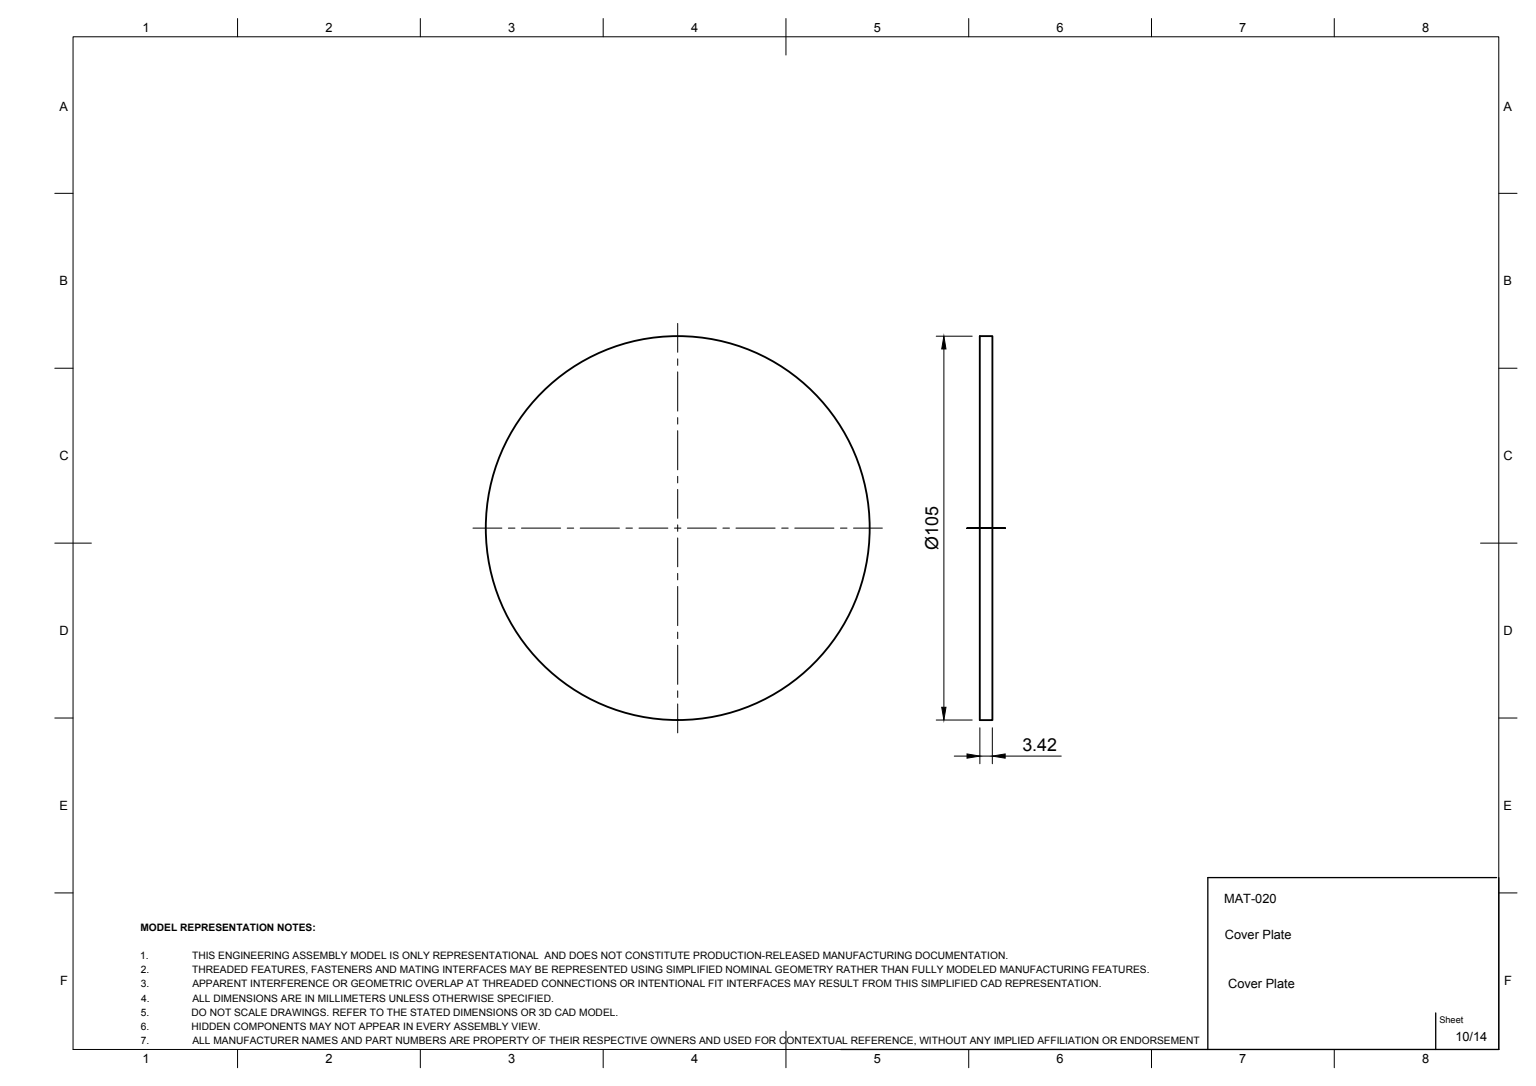
ISO-10303-21;
HEADER;
/* Generated by software containing ST-Developer
 * from STEP Tools, Inc. (www.steptools.com) 
 */

FILE_DESCRIPTION(
/* description */ ('STEP AP214'),
/* implementation_level */ '2;1');

FILE_NAME(
/* name */ 'Cover Plate.step',
/* time_stamp */ '2026-11-14T06:20:50-08:00',
/* author */ (''),
/* organization */ (''),
/* preprocessor_version */ 'ST-DEVELOPER v20.2',
/* originating_system */ 'Autodesk Translation Framework v15.17.0.0',
/* authorisation */ '');

FILE_SCHEMA (('AUTOMOTIVE_DESIGN { 1 0 10303 214 3 1 1 }'));
ENDSEC;

DATA;
#10=MECHANICAL_DESIGN_GEOMETRIC_PRESENTATION_REPRESENTATION('',(#961),#20658);
#422=PLANE('',#3970);
#423=PLANE('',#3971);
#592=LINE('',#20304,#785);
#785=VECTOR('',#4619,52.5);
#905=CYLINDRICAL_SURFACE('',#3967,52.5);
#937=SHAPE_REPRESENTATION_RELATIONSHIP('SRR','None',#20721,#949);
#949=ADVANCED_BREP_SHAPE_REPRESENTATION('',(#973),#20651);
#961=STYLED_ITEM('',(#20786),#973);
#973=MANIFOLD_SOLID_BREP('Body1',#3656);
#1126=FACE_OUTER_BOUND('',#1343,.T.);
#1127=FACE_OUTER_BOUND('',#1344,.T.);
#1128=FACE_OUTER_BOUND('',#1345,.T.);
#1343=EDGE_LOOP('',(#3200,#3201,#3202,#3203));
#1344=EDGE_LOOP('',(#3204));
#1345=EDGE_LOOP('',(#3205));
#1483=CIRCLE('',#3968,52.5);
#1484=CIRCLE('',#3969,52.5);
#1811=VERTEX_POINT('',#20301);
#1812=VERTEX_POINT('',#20303);
#2282=EDGE_CURVE('',#1811,#1811,#1483,.T.);
#2283=EDGE_CURVE('',#1811,#1812,#592,.T.);
#2284=EDGE_CURVE('',#1812,#1812,#1484,.T.);
#3200=ORIENTED_EDGE('',*,*,#2282,.T.);
#3201=ORIENTED_EDGE('',*,*,#2283,.T.);
#3202=ORIENTED_EDGE('',*,*,#2284,.F.);
#3203=ORIENTED_EDGE('',*,*,#2283,.F.);
#3204=ORIENTED_EDGE('',*,*,#2284,.T.);
#3205=ORIENTED_EDGE('',*,*,#2282,.F.);
#3588=ADVANCED_FACE('',(#1126),#905,.T.);
#3589=ADVANCED_FACE('',(#1127),#422,.T.);
#3590=ADVANCED_FACE('',(#1128),#423,.F.);
#3656=CLOSED_SHELL('',(#3588,#3589,#3590));
#3966=AXIS2_PLACEMENT_3D('',#20299,#4613,#4614);
#3967=AXIS2_PLACEMENT_3D('',#20300,#4615,#4616);
#3968=AXIS2_PLACEMENT_3D('',#20302,#4617,#4618);
#3969=AXIS2_PLACEMENT_3D('',#20305,#4620,#4621);
#3970=AXIS2_PLACEMENT_3D('',#20306,#4622,#4623);
#3971=AXIS2_PLACEMENT_3D('',#20307,#4624,#4625);
#4613=DIRECTION('axis',(0.,0.,1.));
#4614=DIRECTION('refdir',(1.,0.,0.));
#4615=DIRECTION('center_axis',(4.93038065763132E-32,2.46519032881566E-32,
-1.));
#4616=DIRECTION('ref_axis',(-1.,-5.55111512312578E-17,-4.93038065763132E-32));
#4617=DIRECTION('center_axis',(-4.93038065763132E-32,-2.46519032881566E-32,
1.));
#4618=DIRECTION('ref_axis',(1.,5.55111512312578E-17,4.93038065763132E-32));
#4619=DIRECTION('',(-4.93038065763132E-32,-2.46519032881566E-32,1.));
#4620=DIRECTION('center_axis',(-4.93038065763132E-32,-2.46519032881566E-32,
1.));
#4621=DIRECTION('ref_axis',(1.,5.55111512312578E-17,4.93038065763132E-32));
#4622=DIRECTION('center_axis',(4.93038065763132E-32,-2.46519032881566E-32,
1.));
#4623=DIRECTION('ref_axis',(1.,5.55111512312578E-17,-4.93038065763132E-32));
#4624=DIRECTION('center_axis',(4.93038065763132E-32,-2.46519032881566E-32,
1.));
#4625=DIRECTION('ref_axis',(1.,5.55111512312578E-17,-4.93038065763132E-32));
#20299=CARTESIAN_POINT('',(0.,0.,0.));
#20300=CARTESIAN_POINT('Origin',(0.,0.,3.42));
#20301=CARTESIAN_POINT('',(52.5,-3.51506025588257E-15,5.55111512312578E-16));
#20302=CARTESIAN_POINT('Origin',(0.,0.,0.));
#20303=CARTESIAN_POINT('',(52.5,-3.51506025588257E-15,3.42));
#20304=CARTESIAN_POINT('',(52.5,-3.51506025588257E-15,3.42));
#20305=CARTESIAN_POINT('Origin',(0.,0.,3.42));
#20306=CARTESIAN_POINT('Origin',(0.,0.,3.42));
#20307=CARTESIAN_POINT('Origin',(0.,0.,0.));
#20637=UNCERTAINTY_MEASURE_WITH_UNIT(LENGTH_MEASURE(0.01),#20659,
'DISTANCE_ACCURACY_VALUE',
'Maximum model space distance between geometric entities at asserted c
onnectivities');
#20644=UNCERTAINTY_MEASURE_WITH_UNIT(LENGTH_MEASURE(0.01),#20659,
'DISTANCE_ACCURACY_VALUE',
'Maximum model space distance between geometric entities at asserted c
onnectivities');
#20651=(
GEOMETRIC_REPRESENTATION_CONTEXT(3)
GLOBAL_UNCERTAINTY_ASSIGNED_CONTEXT((#20637))
GLOBAL_UNIT_ASSIGNED_CONTEXT((#20659,#20661,#20662))
REPRESENTATION_CONTEXT('','3D')
);
#20658=(
GEOMETRIC_REPRESENTATION_CONTEXT(3)
GLOBAL_UNCERTAINTY_ASSIGNED_CONTEXT((#20644))
GLOBAL_UNIT_ASSIGNED_CONTEXT((#20659,#20661,#20662))
REPRESENTATION_CONTEXT('','3D')
);
#20659=(
LENGTH_UNIT()
NAMED_UNIT(*)
SI_UNIT(.MILLI.,.METRE.)
);
#20661=(
NAMED_UNIT(*)
PLANE_ANGLE_UNIT()
SI_UNIT($,.RADIAN.)
);
#20662=(
NAMED_UNIT(*)
SI_UNIT($,.STERADIAN.)
SOLID_ANGLE_UNIT()
);
#20669=SHAPE_DEFINITION_REPRESENTATION(#20682,#20721);
#20682=PRODUCT_DEFINITION_SHAPE('',$,#20735);
#20721=SHAPE_REPRESENTATION('',(#3966),#20651);
#20728=PRODUCT_DEFINITION_CONTEXT('part definition',#20769,'design');
#20735=PRODUCT_DEFINITION('Cover Plate','Cover Plate',#20748,#20728);
#20748=PRODUCT_DEFINITION_FORMATION('',$,#20777);
#20769=APPLICATION_CONTEXT(
'Core Data for Automotive Mechanical Design Process');
#20770=PRODUCT_CONTEXT('part definition',#20769,'mechanical');
#20777=PRODUCT('Cover Plate','Cover Plate',$,(#20770));
#20786=PRESENTATION_STYLE_ASSIGNMENT((#20791));
#20791=SURFACE_STYLE_USAGE(.BOTH.,#20796);
#20796=SURFACE_SIDE_STYLE('',(#20801));
#20801=SURFACE_STYLE_FILL_AREA(#20806);
#20806=FILL_AREA_STYLE('Opaque(61,176,222)',(#20811));
#20811=FILL_AREA_STYLE_COLOUR('Opaque(61,176,222)',#20816);
#20816=COLOUR_RGB('Opaque(61,176,222)',0.23921568627451,0.690196078431373,
0.870588235294118);
ENDSEC;
END-ISO-10303-21;
